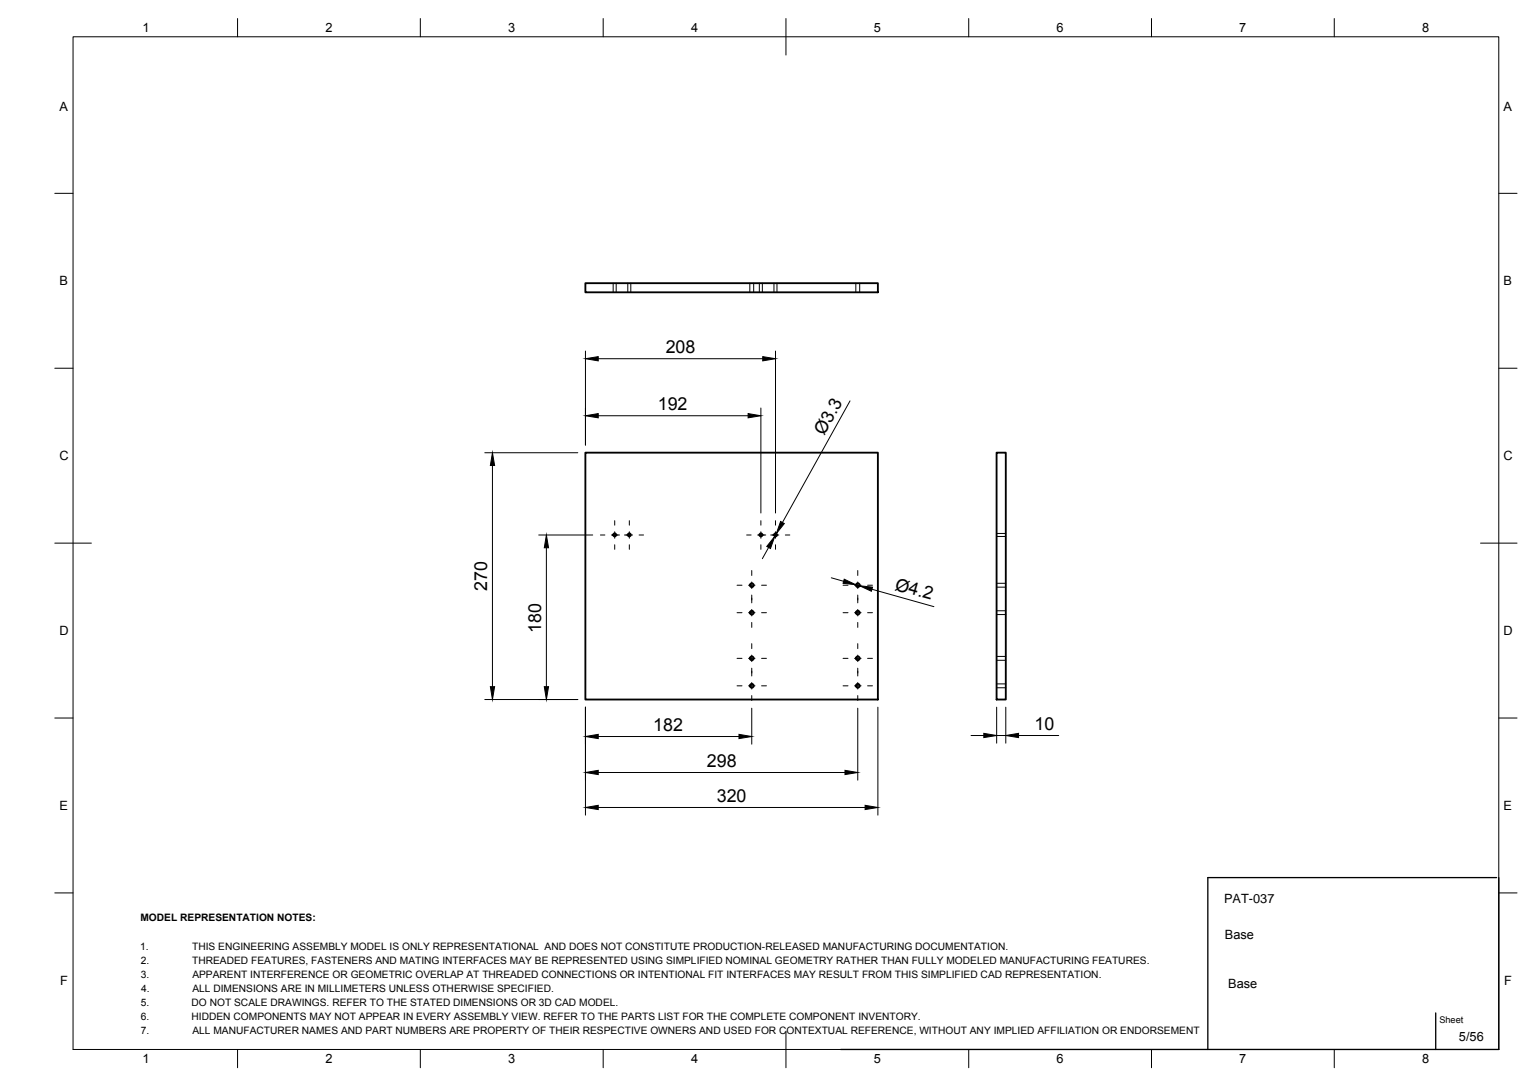
ISO-10303-21;
HEADER;
/* Generated by software containing ST-Developer
 * from STEP Tools, Inc. (www.steptools.com) 
 */

FILE_DESCRIPTION(
/* description */ ('Flywheel Crank-Slider'),
/* implementation_level */ '2;1');

FILE_NAME(
/* name */ 'Base.step',
/* time_stamp */ '2026-10-28T03:23:13-07:00',
/* author */ (''),
/* organization */ (''),
/* preprocessor_version */ 'ST-DEVELOPER v20.2',
/* originating_system */ 'Autodesk Translation Framework v15.17.0.0',
/* authorisation */ '');

FILE_SCHEMA (('AUTOMOTIVE_DESIGN { 1 0 10303 214 3 1 1 }'));
ENDSEC;

DATA;
#10=MECHANICAL_DESIGN_GEOMETRIC_PRESENTATION_REPRESENTATION('',(#668),#17322);
#564=SHAPE_REPRESENTATION_RELATIONSHIP('SRR','None',#17560,#616);
#616=ADVANCED_BREP_SHAPE_REPRESENTATION('',(#729),#17264);
#668=STYLED_ITEM('',(#17910),#729);
#729=MANIFOLD_SOLID_BREP('Body1',#9046);
#785=FACE_BOUND('',#1872,.T.);
#786=FACE_BOUND('',#1873,.T.);
#787=FACE_BOUND('',#1874,.T.);
#788=FACE_BOUND('',#1875,.T.);
#789=FACE_BOUND('',#1876,.T.);
#790=FACE_BOUND('',#1877,.T.);
#791=FACE_BOUND('',#1878,.T.);
#792=FACE_BOUND('',#1879,.T.);
#793=FACE_BOUND('',#1880,.T.);
#794=FACE_BOUND('',#1881,.T.);
#795=FACE_BOUND('',#1882,.T.);
#796=FACE_BOUND('',#1883,.T.);
#797=FACE_BOUND('',#1885,.T.);
#798=FACE_BOUND('',#1886,.T.);
#799=FACE_BOUND('',#1887,.T.);
#800=FACE_BOUND('',#1888,.T.);
#801=FACE_BOUND('',#1889,.T.);
#802=FACE_BOUND('',#1890,.T.);
#803=FACE_BOUND('',#1891,.T.);
#804=FACE_BOUND('',#1892,.T.);
#805=FACE_BOUND('',#1893,.T.);
#806=FACE_BOUND('',#1894,.T.);
#807=FACE_BOUND('',#1895,.T.);
#808=FACE_BOUND('',#1896,.T.);
#1011=PLANE('',#9724);
#1012=PLANE('',#9725);
#1013=PLANE('',#9726);
#1014=PLANE('',#9727);
#1015=PLANE('',#9728);
#1016=PLANE('',#9729);
#1320=FACE_OUTER_BOUND('',#1855,.T.);
#1321=FACE_OUTER_BOUND('',#1856,.T.);
#1322=FACE_OUTER_BOUND('',#1857,.T.);
#1323=FACE_OUTER_BOUND('',#1858,.T.);
#1324=FACE_OUTER_BOUND('',#1859,.T.);
#1325=FACE_OUTER_BOUND('',#1860,.T.);
#1326=FACE_OUTER_BOUND('',#1861,.T.);
#1327=FACE_OUTER_BOUND('',#1862,.T.);
#1328=FACE_OUTER_BOUND('',#1863,.T.);
#1329=FACE_OUTER_BOUND('',#1864,.T.);
#1330=FACE_OUTER_BOUND('',#1865,.T.);
#1331=FACE_OUTER_BOUND('',#1866,.T.);
#1332=FACE_OUTER_BOUND('',#1867,.T.);
#1333=FACE_OUTER_BOUND('',#1868,.T.);
#1334=FACE_OUTER_BOUND('',#1869,.T.);
#1335=FACE_OUTER_BOUND('',#1870,.T.);
#1336=FACE_OUTER_BOUND('',#1871,.T.);
#1337=FACE_OUTER_BOUND('',#1884,.T.);
#1855=EDGE_LOOP('',(#6122,#6123,#6124,#6125));
#1856=EDGE_LOOP('',(#6126,#6127,#6128,#6129));
#1857=EDGE_LOOP('',(#6130,#6131,#6132,#6133));
#1858=EDGE_LOOP('',(#6134,#6135,#6136,#6137));
#1859=EDGE_LOOP('',(#6138,#6139,#6140,#6141));
#1860=EDGE_LOOP('',(#6142,#6143,#6144,#6145));
#1861=EDGE_LOOP('',(#6146,#6147,#6148,#6149));
#1862=EDGE_LOOP('',(#6150,#6151,#6152,#6153));
#1863=EDGE_LOOP('',(#6154,#6155,#6156,#6157));
#1864=EDGE_LOOP('',(#6158,#6159,#6160,#6161));
#1865=EDGE_LOOP('',(#6162,#6163,#6164,#6165));
#1866=EDGE_LOOP('',(#6166,#6167,#6168,#6169));
#1867=EDGE_LOOP('',(#6170,#6171,#6172,#6173));
#1868=EDGE_LOOP('',(#6174,#6175,#6176,#6177));
#1869=EDGE_LOOP('',(#6178,#6179,#6180,#6181));
#1870=EDGE_LOOP('',(#6182,#6183,#6184,#6185));
#1871=EDGE_LOOP('',(#6186,#6187,#6188,#6189));
#1872=EDGE_LOOP('',(#6190));
#1873=EDGE_LOOP('',(#6191));
#1874=EDGE_LOOP('',(#6192));
#1875=EDGE_LOOP('',(#6193));
#1876=EDGE_LOOP('',(#6194));
#1877=EDGE_LOOP('',(#6195));
#1878=EDGE_LOOP('',(#6196));
#1879=EDGE_LOOP('',(#6197));
#1880=EDGE_LOOP('',(#6198));
#1881=EDGE_LOOP('',(#6199));
#1882=EDGE_LOOP('',(#6200));
#1883=EDGE_LOOP('',(#6201));
#1884=EDGE_LOOP('',(#6202,#6203,#6204,#6205));
#1885=EDGE_LOOP('',(#6206));
#1886=EDGE_LOOP('',(#6207));
#1887=EDGE_LOOP('',(#6208));
#1888=EDGE_LOOP('',(#6209));
#1889=EDGE_LOOP('',(#6210));
#1890=EDGE_LOOP('',(#6211));
#1891=EDGE_LOOP('',(#6212));
#1892=EDGE_LOOP('',(#6213));
#1893=EDGE_LOOP('',(#6214));
#1894=EDGE_LOOP('',(#6215));
#1895=EDGE_LOOP('',(#6216));
#1896=EDGE_LOOP('',(#6217));
#2616=LINE('',#13738,#3227);
#2617=LINE('',#13744,#3228);
#2618=LINE('',#13750,#3229);
#2619=LINE('',#13756,#3230);
#2620=LINE('',#13762,#3231);
#2621=LINE('',#13768,#3232);
#2622=LINE('',#13774,#3233);
#2623=LINE('',#13780,#3234);
#2624=LINE('',#13786,#3235);
#2625=LINE('',#13792,#3236);
#2626=LINE('',#13798,#3237);
#2627=LINE('',#13804,#3238);
#2628=LINE('',#13809,#3239);
#2629=LINE('',#13811,#3240);
#2630=LINE('',#13813,#3241);
#2631=LINE('',#13814,#3242);
#2632=LINE('',#13817,#3243);
#2633=LINE('',#13819,#3244);
#2634=LINE('',#13820,#3245);
#2635=LINE('',#13823,#3246);
#2636=LINE('',#13825,#3247);
#2637=LINE('',#13826,#3248);
#2638=LINE('',#13828,#3249);
#2639=LINE('',#13829,#3250);
#3227=VECTOR('',#10840,0.164999999999999);
#3228=VECTOR('',#10847,0.164999999999999);
#3229=VECTOR('',#10854,0.165);
#3230=VECTOR('',#10861,0.165);
#3231=VECTOR('',#10868,0.21);
#3232=VECTOR('',#10875,0.21);
#3233=VECTOR('',#10882,0.21);
#3234=VECTOR('',#10889,0.21);
#3235=VECTOR('',#10896,0.21);
#3236=VECTOR('',#10903,0.21);
#3237=VECTOR('',#10910,0.21);
#3238=VECTOR('',#10917,0.21);
#3239=VECTOR('',#10922,1.);
#3240=VECTOR('',#10923,1.);
#3241=VECTOR('',#10924,1.);
#3242=VECTOR('',#10925,1.);
#3243=VECTOR('',#10928,1.);
#3244=VECTOR('',#10929,1.);
#3245=VECTOR('',#10930,1.);
#3246=VECTOR('',#10933,1.);
#3247=VECTOR('',#10934,1.);
#3248=VECTOR('',#10935,1.);
#3249=VECTOR('',#10938,1.);
#3250=VECTOR('',#10939,1.);
#3838=CIRCLE('',#9689,0.164999999999999);
#3839=CIRCLE('',#9690,0.164999999999999);
#3840=CIRCLE('',#9692,0.164999999999999);
#3841=CIRCLE('',#9693,0.164999999999999);
#3842=CIRCLE('',#9695,0.165);
#3843=CIRCLE('',#9696,0.165);
#3844=CIRCLE('',#9698,0.165);
#3845=CIRCLE('',#9699,0.165);
#3846=CIRCLE('',#9701,0.21);
#3847=CIRCLE('',#9702,0.21);
#3848=CIRCLE('',#9704,0.21);
#3849=CIRCLE('',#9705,0.21);
#3850=CIRCLE('',#9707,0.21);
#3851=CIRCLE('',#9708,0.21);
#3852=CIRCLE('',#9710,0.21);
#3853=CIRCLE('',#9711,0.21);
#3854=CIRCLE('',#9713,0.21);
#3855=CIRCLE('',#9714,0.21);
#3856=CIRCLE('',#9716,0.21);
#3857=CIRCLE('',#9717,0.21);
#3858=CIRCLE('',#9719,0.21);
#3859=CIRCLE('',#9720,0.21);
#3860=CIRCLE('',#9722,0.21);
#3861=CIRCLE('',#9723,0.21);
#4277=VERTEX_POINT('',#13735);
#4278=VERTEX_POINT('',#13737);
#4279=VERTEX_POINT('',#13741);
#4280=VERTEX_POINT('',#13743);
#4281=VERTEX_POINT('',#13747);
#4282=VERTEX_POINT('',#13749);
#4283=VERTEX_POINT('',#13753);
#4284=VERTEX_POINT('',#13755);
#4285=VERTEX_POINT('',#13759);
#4286=VERTEX_POINT('',#13761);
#4287=VERTEX_POINT('',#13765);
#4288=VERTEX_POINT('',#13767);
#4289=VERTEX_POINT('',#13771);
#4290=VERTEX_POINT('',#13773);
#4291=VERTEX_POINT('',#13777);
#4292=VERTEX_POINT('',#13779);
#4293=VERTEX_POINT('',#13783);
#4294=VERTEX_POINT('',#13785);
#4295=VERTEX_POINT('',#13789);
#4296=VERTEX_POINT('',#13791);
#4297=VERTEX_POINT('',#13795);
#4298=VERTEX_POINT('',#13797);
#4299=VERTEX_POINT('',#13801);
#4300=VERTEX_POINT('',#13803);
#4301=VERTEX_POINT('',#13807);
#4302=VERTEX_POINT('',#13808);
#4303=VERTEX_POINT('',#13810);
#4304=VERTEX_POINT('',#13812);
#4305=VERTEX_POINT('',#13816);
#4306=VERTEX_POINT('',#13818);
#4307=VERTEX_POINT('',#13822);
#4308=VERTEX_POINT('',#13824);
#5018=EDGE_CURVE('',#4277,#4277,#3838,.T.);
#5019=EDGE_CURVE('',#4277,#4278,#2616,.T.);
#5020=EDGE_CURVE('',#4278,#4278,#3839,.T.);
#5021=EDGE_CURVE('',#4279,#4279,#3840,.T.);
#5022=EDGE_CURVE('',#4279,#4280,#2617,.T.);
#5023=EDGE_CURVE('',#4280,#4280,#3841,.T.);
#5024=EDGE_CURVE('',#4281,#4281,#3842,.T.);
#5025=EDGE_CURVE('',#4281,#4282,#2618,.T.);
#5026=EDGE_CURVE('',#4282,#4282,#3843,.T.);
#5027=EDGE_CURVE('',#4283,#4283,#3844,.T.);
#5028=EDGE_CURVE('',#4283,#4284,#2619,.T.);
#5029=EDGE_CURVE('',#4284,#4284,#3845,.T.);
#5030=EDGE_CURVE('',#4285,#4285,#3846,.T.);
#5031=EDGE_CURVE('',#4285,#4286,#2620,.T.);
#5032=EDGE_CURVE('',#4286,#4286,#3847,.T.);
#5033=EDGE_CURVE('',#4287,#4287,#3848,.T.);
#5034=EDGE_CURVE('',#4287,#4288,#2621,.T.);
#5035=EDGE_CURVE('',#4288,#4288,#3849,.T.);
#5036=EDGE_CURVE('',#4289,#4289,#3850,.T.);
#5037=EDGE_CURVE('',#4289,#4290,#2622,.T.);
#5038=EDGE_CURVE('',#4290,#4290,#3851,.T.);
#5039=EDGE_CURVE('',#4291,#4291,#3852,.T.);
#5040=EDGE_CURVE('',#4291,#4292,#2623,.T.);
#5041=EDGE_CURVE('',#4292,#4292,#3853,.T.);
#5042=EDGE_CURVE('',#4293,#4293,#3854,.T.);
#5043=EDGE_CURVE('',#4293,#4294,#2624,.T.);
#5044=EDGE_CURVE('',#4294,#4294,#3855,.T.);
#5045=EDGE_CURVE('',#4295,#4295,#3856,.T.);
#5046=EDGE_CURVE('',#4295,#4296,#2625,.T.);
#5047=EDGE_CURVE('',#4296,#4296,#3857,.T.);
#5048=EDGE_CURVE('',#4297,#4297,#3858,.T.);
#5049=EDGE_CURVE('',#4297,#4298,#2626,.T.);
#5050=EDGE_CURVE('',#4298,#4298,#3859,.T.);
#5051=EDGE_CURVE('',#4299,#4299,#3860,.T.);
#5052=EDGE_CURVE('',#4299,#4300,#2627,.T.);
#5053=EDGE_CURVE('',#4300,#4300,#3861,.T.);
#5054=EDGE_CURVE('',#4301,#4302,#2628,.T.);
#5055=EDGE_CURVE('',#4302,#4303,#2629,.T.);
#5056=EDGE_CURVE('',#4304,#4303,#2630,.T.);
#5057=EDGE_CURVE('',#4301,#4304,#2631,.T.);
#5058=EDGE_CURVE('',#4305,#4301,#2632,.T.);
#5059=EDGE_CURVE('',#4306,#4304,#2633,.T.);
#5060=EDGE_CURVE('',#4305,#4306,#2634,.T.);
#5061=EDGE_CURVE('',#4307,#4305,#2635,.T.);
#5062=EDGE_CURVE('',#4308,#4306,#2636,.T.);
#5063=EDGE_CURVE('',#4307,#4308,#2637,.T.);
#5064=EDGE_CURVE('',#4302,#4307,#2638,.T.);
#5065=EDGE_CURVE('',#4303,#4308,#2639,.T.);
#6122=ORIENTED_EDGE('',*,*,#5018,.F.);
#6123=ORIENTED_EDGE('',*,*,#5019,.T.);
#6124=ORIENTED_EDGE('',*,*,#5020,.F.);
#6125=ORIENTED_EDGE('',*,*,#5019,.F.);
#6126=ORIENTED_EDGE('',*,*,#5021,.F.);
#6127=ORIENTED_EDGE('',*,*,#5022,.T.);
#6128=ORIENTED_EDGE('',*,*,#5023,.F.);
#6129=ORIENTED_EDGE('',*,*,#5022,.F.);
#6130=ORIENTED_EDGE('',*,*,#5024,.F.);
#6131=ORIENTED_EDGE('',*,*,#5025,.T.);
#6132=ORIENTED_EDGE('',*,*,#5026,.F.);
#6133=ORIENTED_EDGE('',*,*,#5025,.F.);
#6134=ORIENTED_EDGE('',*,*,#5027,.F.);
#6135=ORIENTED_EDGE('',*,*,#5028,.T.);
#6136=ORIENTED_EDGE('',*,*,#5029,.F.);
#6137=ORIENTED_EDGE('',*,*,#5028,.F.);
#6138=ORIENTED_EDGE('',*,*,#5030,.F.);
#6139=ORIENTED_EDGE('',*,*,#5031,.T.);
#6140=ORIENTED_EDGE('',*,*,#5032,.F.);
#6141=ORIENTED_EDGE('',*,*,#5031,.F.);
#6142=ORIENTED_EDGE('',*,*,#5033,.F.);
#6143=ORIENTED_EDGE('',*,*,#5034,.T.);
#6144=ORIENTED_EDGE('',*,*,#5035,.F.);
#6145=ORIENTED_EDGE('',*,*,#5034,.F.);
#6146=ORIENTED_EDGE('',*,*,#5036,.F.);
#6147=ORIENTED_EDGE('',*,*,#5037,.T.);
#6148=ORIENTED_EDGE('',*,*,#5038,.F.);
#6149=ORIENTED_EDGE('',*,*,#5037,.F.);
#6150=ORIENTED_EDGE('',*,*,#5039,.F.);
#6151=ORIENTED_EDGE('',*,*,#5040,.T.);
#6152=ORIENTED_EDGE('',*,*,#5041,.F.);
#6153=ORIENTED_EDGE('',*,*,#5040,.F.);
#6154=ORIENTED_EDGE('',*,*,#5042,.F.);
#6155=ORIENTED_EDGE('',*,*,#5043,.T.);
#6156=ORIENTED_EDGE('',*,*,#5044,.F.);
#6157=ORIENTED_EDGE('',*,*,#5043,.F.);
#6158=ORIENTED_EDGE('',*,*,#5045,.F.);
#6159=ORIENTED_EDGE('',*,*,#5046,.T.);
#6160=ORIENTED_EDGE('',*,*,#5047,.F.);
#6161=ORIENTED_EDGE('',*,*,#5046,.F.);
#6162=ORIENTED_EDGE('',*,*,#5048,.F.);
#6163=ORIENTED_EDGE('',*,*,#5049,.T.);
#6164=ORIENTED_EDGE('',*,*,#5050,.F.);
#6165=ORIENTED_EDGE('',*,*,#5049,.F.);
#6166=ORIENTED_EDGE('',*,*,#5051,.F.);
#6167=ORIENTED_EDGE('',*,*,#5052,.T.);
#6168=ORIENTED_EDGE('',*,*,#5053,.F.);
#6169=ORIENTED_EDGE('',*,*,#5052,.F.);
#6170=ORIENTED_EDGE('',*,*,#5054,.T.);
#6171=ORIENTED_EDGE('',*,*,#5055,.T.);
#6172=ORIENTED_EDGE('',*,*,#5056,.F.);
#6173=ORIENTED_EDGE('',*,*,#5057,.F.);
#6174=ORIENTED_EDGE('',*,*,#5058,.T.);
#6175=ORIENTED_EDGE('',*,*,#5057,.T.);
#6176=ORIENTED_EDGE('',*,*,#5059,.F.);
#6177=ORIENTED_EDGE('',*,*,#5060,.F.);
#6178=ORIENTED_EDGE('',*,*,#5061,.T.);
#6179=ORIENTED_EDGE('',*,*,#5060,.T.);
#6180=ORIENTED_EDGE('',*,*,#5062,.F.);
#6181=ORIENTED_EDGE('',*,*,#5063,.F.);
#6182=ORIENTED_EDGE('',*,*,#5064,.T.);
#6183=ORIENTED_EDGE('',*,*,#5063,.T.);
#6184=ORIENTED_EDGE('',*,*,#5065,.F.);
#6185=ORIENTED_EDGE('',*,*,#5055,.F.);
#6186=ORIENTED_EDGE('',*,*,#5065,.T.);
#6187=ORIENTED_EDGE('',*,*,#5062,.T.);
#6188=ORIENTED_EDGE('',*,*,#5059,.T.);
#6189=ORIENTED_EDGE('',*,*,#5056,.T.);
#6190=ORIENTED_EDGE('',*,*,#5026,.T.);
#6191=ORIENTED_EDGE('',*,*,#5029,.T.);
#6192=ORIENTED_EDGE('',*,*,#5053,.T.);
#6193=ORIENTED_EDGE('',*,*,#5050,.T.);
#6194=ORIENTED_EDGE('',*,*,#5047,.T.);
#6195=ORIENTED_EDGE('',*,*,#5044,.T.);
#6196=ORIENTED_EDGE('',*,*,#5041,.T.);
#6197=ORIENTED_EDGE('',*,*,#5038,.T.);
#6198=ORIENTED_EDGE('',*,*,#5035,.T.);
#6199=ORIENTED_EDGE('',*,*,#5032,.T.);
#6200=ORIENTED_EDGE('',*,*,#5023,.T.);
#6201=ORIENTED_EDGE('',*,*,#5020,.T.);
#6202=ORIENTED_EDGE('',*,*,#5064,.F.);
#6203=ORIENTED_EDGE('',*,*,#5054,.F.);
#6204=ORIENTED_EDGE('',*,*,#5058,.F.);
#6205=ORIENTED_EDGE('',*,*,#5061,.F.);
#6206=ORIENTED_EDGE('',*,*,#5024,.T.);
#6207=ORIENTED_EDGE('',*,*,#5027,.T.);
#6208=ORIENTED_EDGE('',*,*,#5051,.T.);
#6209=ORIENTED_EDGE('',*,*,#5048,.T.);
#6210=ORIENTED_EDGE('',*,*,#5045,.T.);
#6211=ORIENTED_EDGE('',*,*,#5042,.T.);
#6212=ORIENTED_EDGE('',*,*,#5039,.T.);
#6213=ORIENTED_EDGE('',*,*,#5036,.T.);
#6214=ORIENTED_EDGE('',*,*,#5033,.T.);
#6215=ORIENTED_EDGE('',*,*,#5030,.T.);
#6216=ORIENTED_EDGE('',*,*,#5021,.T.);
#6217=ORIENTED_EDGE('',*,*,#5018,.T.);
#8330=CYLINDRICAL_SURFACE('',#9688,0.164999999999999);
#8331=CYLINDRICAL_SURFACE('',#9691,0.164999999999999);
#8332=CYLINDRICAL_SURFACE('',#9694,0.165);
#8333=CYLINDRICAL_SURFACE('',#9697,0.165);
#8334=CYLINDRICAL_SURFACE('',#9700,0.21);
#8335=CYLINDRICAL_SURFACE('',#9703,0.21);
#8336=CYLINDRICAL_SURFACE('',#9706,0.21);
#8337=CYLINDRICAL_SURFACE('',#9709,0.21);
#8338=CYLINDRICAL_SURFACE('',#9712,0.21);
#8339=CYLINDRICAL_SURFACE('',#9715,0.21);
#8340=CYLINDRICAL_SURFACE('',#9718,0.21);
#8341=CYLINDRICAL_SURFACE('',#9721,0.21);
#8511=ADVANCED_FACE('',(#1320),#8330,.F.);
#8512=ADVANCED_FACE('',(#1321),#8331,.F.);
#8513=ADVANCED_FACE('',(#1322),#8332,.F.);
#8514=ADVANCED_FACE('',(#1323),#8333,.F.);
#8515=ADVANCED_FACE('',(#1324),#8334,.F.);
#8516=ADVANCED_FACE('',(#1325),#8335,.F.);
#8517=ADVANCED_FACE('',(#1326),#8336,.F.);
#8518=ADVANCED_FACE('',(#1327),#8337,.F.);
#8519=ADVANCED_FACE('',(#1328),#8338,.F.);
#8520=ADVANCED_FACE('',(#1329),#8339,.F.);
#8521=ADVANCED_FACE('',(#1330),#8340,.F.);
#8522=ADVANCED_FACE('',(#1331),#8341,.F.);
#8523=ADVANCED_FACE('',(#1332),#1011,.T.);
#8524=ADVANCED_FACE('',(#1333),#1012,.T.);
#8525=ADVANCED_FACE('',(#1334),#1013,.T.);
#8526=ADVANCED_FACE('',(#1335),#1014,.T.);
#8527=ADVANCED_FACE('',(#1336,#785,#786,#787,#788,#789,#790,#791,#792,#793,
#794,#795,#796),#1015,.T.);
#8528=ADVANCED_FACE('',(#1337,#797,#798,#799,#800,#801,#802,#803,#804,#805,
#806,#807,#808),#1016,.F.);
#9046=CLOSED_SHELL('',(#8511,#8512,#8513,#8514,#8515,#8516,#8517,#8518,
#8519,#8520,#8521,#8522,#8523,#8524,#8525,#8526,#8527,#8528));
#9687=AXIS2_PLACEMENT_3D('',#13733,#10834,#10835);
#9688=AXIS2_PLACEMENT_3D('',#13734,#10836,#10837);
#9689=AXIS2_PLACEMENT_3D('',#13736,#10838,#10839);
#9690=AXIS2_PLACEMENT_3D('',#13739,#10841,#10842);
#9691=AXIS2_PLACEMENT_3D('',#13740,#10843,#10844);
#9692=AXIS2_PLACEMENT_3D('',#13742,#10845,#10846);
#9693=AXIS2_PLACEMENT_3D('',#13745,#10848,#10849);
#9694=AXIS2_PLACEMENT_3D('',#13746,#10850,#10851);
#9695=AXIS2_PLACEMENT_3D('',#13748,#10852,#10853);
#9696=AXIS2_PLACEMENT_3D('',#13751,#10855,#10856);
#9697=AXIS2_PLACEMENT_3D('',#13752,#10857,#10858);
#9698=AXIS2_PLACEMENT_3D('',#13754,#10859,#10860);
#9699=AXIS2_PLACEMENT_3D('',#13757,#10862,#10863);
#9700=AXIS2_PLACEMENT_3D('',#13758,#10864,#10865);
#9701=AXIS2_PLACEMENT_3D('',#13760,#10866,#10867);
#9702=AXIS2_PLACEMENT_3D('',#13763,#10869,#10870);
#9703=AXIS2_PLACEMENT_3D('',#13764,#10871,#10872);
#9704=AXIS2_PLACEMENT_3D('',#13766,#10873,#10874);
#9705=AXIS2_PLACEMENT_3D('',#13769,#10876,#10877);
#9706=AXIS2_PLACEMENT_3D('',#13770,#10878,#10879);
#9707=AXIS2_PLACEMENT_3D('',#13772,#10880,#10881);
#9708=AXIS2_PLACEMENT_3D('',#13775,#10883,#10884);
#9709=AXIS2_PLACEMENT_3D('',#13776,#10885,#10886);
#9710=AXIS2_PLACEMENT_3D('',#13778,#10887,#10888);
#9711=AXIS2_PLACEMENT_3D('',#13781,#10890,#10891);
#9712=AXIS2_PLACEMENT_3D('',#13782,#10892,#10893);
#9713=AXIS2_PLACEMENT_3D('',#13784,#10894,#10895);
#9714=AXIS2_PLACEMENT_3D('',#13787,#10897,#10898);
#9715=AXIS2_PLACEMENT_3D('',#13788,#10899,#10900);
#9716=AXIS2_PLACEMENT_3D('',#13790,#10901,#10902);
#9717=AXIS2_PLACEMENT_3D('',#13793,#10904,#10905);
#9718=AXIS2_PLACEMENT_3D('',#13794,#10906,#10907);
#9719=AXIS2_PLACEMENT_3D('',#13796,#10908,#10909);
#9720=AXIS2_PLACEMENT_3D('',#13799,#10911,#10912);
#9721=AXIS2_PLACEMENT_3D('',#13800,#10913,#10914);
#9722=AXIS2_PLACEMENT_3D('',#13802,#10915,#10916);
#9723=AXIS2_PLACEMENT_3D('',#13805,#10918,#10919);
#9724=AXIS2_PLACEMENT_3D('',#13806,#10920,#10921);
#9725=AXIS2_PLACEMENT_3D('',#13815,#10926,#10927);
#9726=AXIS2_PLACEMENT_3D('',#13821,#10931,#10932);
#9727=AXIS2_PLACEMENT_3D('',#13827,#10936,#10937);
#9728=AXIS2_PLACEMENT_3D('',#13830,#10940,#10941);
#9729=AXIS2_PLACEMENT_3D('',#13831,#10942,#10943);
#10834=DIRECTION('axis',(0.,0.,1.));
#10835=DIRECTION('refdir',(1.,0.,0.));
#10836=DIRECTION('center_axis',(0.,0.,1.));
#10837=DIRECTION('ref_axis',(1.,0.,0.));
#10838=DIRECTION('center_axis',(0.,0.,1.));
#10839=DIRECTION('ref_axis',(1.,0.,0.));
#10840=DIRECTION('',(0.,0.,1.));
#10841=DIRECTION('center_axis',(0.,0.,-1.));
#10842=DIRECTION('ref_axis',(1.,0.,0.));
#10843=DIRECTION('center_axis',(0.,0.,1.));
#10844=DIRECTION('ref_axis',(1.,0.,0.));
#10845=DIRECTION('center_axis',(0.,0.,1.));
#10846=DIRECTION('ref_axis',(1.,0.,0.));
#10847=DIRECTION('',(0.,0.,1.));
#10848=DIRECTION('center_axis',(0.,0.,-1.));
#10849=DIRECTION('ref_axis',(1.,0.,0.));
#10850=DIRECTION('center_axis',(0.,0.,1.));
#10851=DIRECTION('ref_axis',(1.,0.,0.));
#10852=DIRECTION('center_axis',(0.,0.,1.));
#10853=DIRECTION('ref_axis',(1.,0.,0.));
#10854=DIRECTION('',(0.,0.,1.));
#10855=DIRECTION('center_axis',(0.,0.,-1.));
#10856=DIRECTION('ref_axis',(1.,0.,0.));
#10857=DIRECTION('center_axis',(0.,0.,1.));
#10858=DIRECTION('ref_axis',(1.,0.,0.));
#10859=DIRECTION('center_axis',(0.,0.,1.));
#10860=DIRECTION('ref_axis',(1.,0.,0.));
#10861=DIRECTION('',(0.,0.,1.));
#10862=DIRECTION('center_axis',(0.,0.,-1.));
#10863=DIRECTION('ref_axis',(1.,0.,0.));
#10864=DIRECTION('center_axis',(0.,0.,1.));
#10865=DIRECTION('ref_axis',(1.,0.,0.));
#10866=DIRECTION('center_axis',(0.,0.,1.));
#10867=DIRECTION('ref_axis',(1.,0.,0.));
#10868=DIRECTION('',(0.,0.,1.));
#10869=DIRECTION('center_axis',(0.,0.,-1.));
#10870=DIRECTION('ref_axis',(1.,0.,0.));
#10871=DIRECTION('center_axis',(0.,0.,1.));
#10872=DIRECTION('ref_axis',(1.,0.,0.));
#10873=DIRECTION('center_axis',(0.,0.,1.));
#10874=DIRECTION('ref_axis',(1.,0.,0.));
#10875=DIRECTION('',(0.,0.,1.));
#10876=DIRECTION('center_axis',(0.,0.,-1.));
#10877=DIRECTION('ref_axis',(1.,0.,0.));
#10878=DIRECTION('center_axis',(0.,0.,1.));
#10879=DIRECTION('ref_axis',(1.,0.,0.));
#10880=DIRECTION('center_axis',(0.,0.,1.));
#10881=DIRECTION('ref_axis',(1.,0.,0.));
#10882=DIRECTION('',(0.,0.,1.));
#10883=DIRECTION('center_axis',(0.,0.,-1.));
#10884=DIRECTION('ref_axis',(1.,0.,0.));
#10885=DIRECTION('center_axis',(0.,0.,1.));
#10886=DIRECTION('ref_axis',(1.,0.,0.));
#10887=DIRECTION('center_axis',(0.,0.,1.));
#10888=DIRECTION('ref_axis',(1.,0.,0.));
#10889=DIRECTION('',(0.,0.,1.));
#10890=DIRECTION('center_axis',(0.,0.,-1.));
#10891=DIRECTION('ref_axis',(1.,0.,0.));
#10892=DIRECTION('center_axis',(0.,0.,1.));
#10893=DIRECTION('ref_axis',(1.,0.,0.));
#10894=DIRECTION('center_axis',(0.,0.,1.));
#10895=DIRECTION('ref_axis',(1.,0.,0.));
#10896=DIRECTION('',(0.,0.,1.));
#10897=DIRECTION('center_axis',(0.,0.,-1.));
#10898=DIRECTION('ref_axis',(1.,0.,0.));
#10899=DIRECTION('center_axis',(0.,0.,1.));
#10900=DIRECTION('ref_axis',(1.,0.,0.));
#10901=DIRECTION('center_axis',(0.,0.,1.));
#10902=DIRECTION('ref_axis',(1.,0.,0.));
#10903=DIRECTION('',(0.,0.,1.));
#10904=DIRECTION('center_axis',(0.,0.,-1.));
#10905=DIRECTION('ref_axis',(1.,0.,0.));
#10906=DIRECTION('center_axis',(0.,0.,1.));
#10907=DIRECTION('ref_axis',(1.,0.,0.));
#10908=DIRECTION('center_axis',(0.,0.,1.));
#10909=DIRECTION('ref_axis',(1.,0.,0.));
#10910=DIRECTION('',(0.,0.,1.));
#10911=DIRECTION('center_axis',(0.,0.,-1.));
#10912=DIRECTION('ref_axis',(1.,0.,0.));
#10913=DIRECTION('center_axis',(0.,0.,1.));
#10914=DIRECTION('ref_axis',(1.,0.,0.));
#10915=DIRECTION('center_axis',(0.,0.,1.));
#10916=DIRECTION('ref_axis',(1.,0.,0.));
#10917=DIRECTION('',(0.,0.,1.));
#10918=DIRECTION('center_axis',(0.,0.,-1.));
#10919=DIRECTION('ref_axis',(1.,0.,0.));
#10920=DIRECTION('center_axis',(0.,1.,0.));
#10921=DIRECTION('ref_axis',(-1.,0.,0.));
#10922=DIRECTION('',(-1.,0.,0.));
#10923=DIRECTION('',(0.,0.,1.));
#10924=DIRECTION('',(-1.,0.,0.));
#10925=DIRECTION('',(0.,0.,1.));
#10926=DIRECTION('center_axis',(1.,0.,0.));
#10927=DIRECTION('ref_axis',(0.,1.,0.));
#10928=DIRECTION('',(0.,1.,0.));
#10929=DIRECTION('',(0.,1.,0.));
#10930=DIRECTION('',(0.,0.,1.));
#10931=DIRECTION('center_axis',(0.,-1.,0.));
#10932=DIRECTION('ref_axis',(1.,0.,0.));
#10933=DIRECTION('',(1.,0.,0.));
#10934=DIRECTION('',(1.,0.,0.));
#10935=DIRECTION('',(0.,0.,1.));
#10936=DIRECTION('center_axis',(-1.,0.,0.));
#10937=DIRECTION('ref_axis',(0.,-1.,0.));
#10938=DIRECTION('',(0.,-1.,0.));
#10939=DIRECTION('',(0.,-1.,0.));
#10940=DIRECTION('center_axis',(0.,0.,1.));
#10941=DIRECTION('ref_axis',(1.,0.,0.));
#10942=DIRECTION('center_axis',(0.,0.,1.));
#10943=DIRECTION('ref_axis',(1.,0.,0.));
#13733=CARTESIAN_POINT('',(0.,0.,0.));
#13734=CARTESIAN_POINT('Origin',(19.2,0.,-0.1));
#13735=CARTESIAN_POINT('',(19.035,-2.02066721859312E-17,0.));
#13736=CARTESIAN_POINT('Origin',(19.2,0.,0.));
#13737=CARTESIAN_POINT('',(19.035,2.02066721859312E-17,1.));
#13738=CARTESIAN_POINT('',(19.035,-2.02066721859312E-17,-0.1));
#13739=CARTESIAN_POINT('Origin',(19.2,0.,1.));
#13740=CARTESIAN_POINT('Origin',(20.8,0.,-0.1));
#13741=CARTESIAN_POINT('',(20.635,-2.02066721859312E-17,0.));
#13742=CARTESIAN_POINT('Origin',(20.8,0.,0.));
#13743=CARTESIAN_POINT('',(20.635,2.02066721859312E-17,1.));
#13744=CARTESIAN_POINT('',(20.635,-2.02066721859312E-17,-0.1));
#13745=CARTESIAN_POINT('Origin',(20.8,0.,1.));
#13746=CARTESIAN_POINT('Origin',(3.2,0.,-0.1));
#13747=CARTESIAN_POINT('',(3.035,-2.02066721859313E-17,0.));
#13748=CARTESIAN_POINT('Origin',(3.2,0.,0.));
#13749=CARTESIAN_POINT('',(3.035,2.02066721859313E-17,1.));
#13750=CARTESIAN_POINT('',(3.035,-2.02066721859313E-17,-0.1));
#13751=CARTESIAN_POINT('Origin',(3.2,0.,1.));
#13752=CARTESIAN_POINT('Origin',(4.8,0.,-0.1));
#13753=CARTESIAN_POINT('',(4.635,-2.02066721859313E-17,0.));
#13754=CARTESIAN_POINT('Origin',(4.8,0.,0.));
#13755=CARTESIAN_POINT('',(4.635,2.02066721859313E-17,1.));
#13756=CARTESIAN_POINT('',(4.635,-2.02066721859313E-17,-0.1));
#13757=CARTESIAN_POINT('Origin',(4.8,0.,1.));
#13758=CARTESIAN_POINT('Origin',(5.8,-8.5,-0.1));
#13759=CARTESIAN_POINT('',(5.59,-8.5,0.));
#13760=CARTESIAN_POINT('Origin',(5.8,-8.5,0.));
#13761=CARTESIAN_POINT('',(5.59,-8.5,1.));
#13762=CARTESIAN_POINT('',(5.59,-8.5,-0.1));
#13763=CARTESIAN_POINT('Origin',(5.8,-8.5,1.));
#13764=CARTESIAN_POINT('Origin',(-5.8,-5.5,-0.1));
#13765=CARTESIAN_POINT('',(-6.01,-5.5,0.));
#13766=CARTESIAN_POINT('Origin',(-5.8,-5.5,0.));
#13767=CARTESIAN_POINT('',(-6.01,-5.5,1.));
#13768=CARTESIAN_POINT('',(-6.01,-5.5,-0.1));
#13769=CARTESIAN_POINT('Origin',(-5.8,-5.5,1.));
#13770=CARTESIAN_POINT('Origin',(-5.8,-8.5,-0.1));
#13771=CARTESIAN_POINT('',(-6.01,-8.5,0.));
#13772=CARTESIAN_POINT('Origin',(-5.8,-8.5,0.));
#13773=CARTESIAN_POINT('',(-6.01,-8.5,1.));
#13774=CARTESIAN_POINT('',(-6.01,-8.5,-0.1));
#13775=CARTESIAN_POINT('Origin',(-5.8,-8.5,1.));
#13776=CARTESIAN_POINT('Origin',(5.8,-5.5,-0.1));
#13777=CARTESIAN_POINT('',(5.59,-5.5,0.));
#13778=CARTESIAN_POINT('Origin',(5.8,-5.5,0.));
#13779=CARTESIAN_POINT('',(5.59,-5.5,1.));
#13780=CARTESIAN_POINT('',(5.59,-5.5,-0.1));
#13781=CARTESIAN_POINT('Origin',(5.8,-5.5,1.));
#13782=CARTESIAN_POINT('Origin',(5.8,-16.5,-0.1));
#13783=CARTESIAN_POINT('',(5.59,-16.5,0.));
#13784=CARTESIAN_POINT('Origin',(5.8,-16.5,0.));
#13785=CARTESIAN_POINT('',(5.59,-16.5,1.));
#13786=CARTESIAN_POINT('',(5.59,-16.5,-0.1));
#13787=CARTESIAN_POINT('Origin',(5.8,-16.5,1.));
#13788=CARTESIAN_POINT('Origin',(-5.8,-13.5,-0.1));
#13789=CARTESIAN_POINT('',(-6.01,-13.5,0.));
#13790=CARTESIAN_POINT('Origin',(-5.8,-13.5,0.));
#13791=CARTESIAN_POINT('',(-6.01,-13.5,1.));
#13792=CARTESIAN_POINT('',(-6.01,-13.5,-0.1));
#13793=CARTESIAN_POINT('Origin',(-5.8,-13.5,1.));
#13794=CARTESIAN_POINT('Origin',(-5.8,-16.5,-0.1));
#13795=CARTESIAN_POINT('',(-6.01,-16.5,0.));
#13796=CARTESIAN_POINT('Origin',(-5.8,-16.5,0.));
#13797=CARTESIAN_POINT('',(-6.01,-16.5,1.));
#13798=CARTESIAN_POINT('',(-6.01,-16.5,-0.1));
#13799=CARTESIAN_POINT('Origin',(-5.8,-16.5,1.));
#13800=CARTESIAN_POINT('Origin',(5.8,-13.5,-0.1));
#13801=CARTESIAN_POINT('',(5.59,-13.5,0.));
#13802=CARTESIAN_POINT('Origin',(5.8,-13.5,0.));
#13803=CARTESIAN_POINT('',(5.59,-13.5,1.));
#13804=CARTESIAN_POINT('',(5.59,-13.5,-0.1));
#13805=CARTESIAN_POINT('Origin',(5.8,-13.5,1.));
#13806=CARTESIAN_POINT('Origin',(24.,9.,0.));
#13807=CARTESIAN_POINT('',(24.,9.,0.));
#13808=CARTESIAN_POINT('',(-8.,9.,0.));
#13809=CARTESIAN_POINT('',(24.,9.,0.));
#13810=CARTESIAN_POINT('',(-8.,9.,1.));
#13811=CARTESIAN_POINT('',(-8.,9.,0.));
#13812=CARTESIAN_POINT('',(24.,9.,1.));
#13813=CARTESIAN_POINT('',(24.,9.,1.));
#13814=CARTESIAN_POINT('',(24.,9.,0.));
#13815=CARTESIAN_POINT('Origin',(24.,-18.,0.));
#13816=CARTESIAN_POINT('',(24.,-18.,0.));
#13817=CARTESIAN_POINT('',(24.,-18.,0.));
#13818=CARTESIAN_POINT('',(24.,-18.,1.));
#13819=CARTESIAN_POINT('',(24.,-18.,1.));
#13820=CARTESIAN_POINT('',(24.,-18.,0.));
#13821=CARTESIAN_POINT('Origin',(-8.,-18.,0.));
#13822=CARTESIAN_POINT('',(-8.,-18.,0.));
#13823=CARTESIAN_POINT('',(-8.,-18.,0.));
#13824=CARTESIAN_POINT('',(-8.,-18.,1.));
#13825=CARTESIAN_POINT('',(-8.,-18.,1.));
#13826=CARTESIAN_POINT('',(-8.,-18.,0.));
#13827=CARTESIAN_POINT('Origin',(-8.,9.,0.));
#13828=CARTESIAN_POINT('',(-8.,9.,0.));
#13829=CARTESIAN_POINT('',(-8.,9.,1.));
#13830=CARTESIAN_POINT('Origin',(8.,-4.5,1.));
#13831=CARTESIAN_POINT('Origin',(8.,-4.5,0.));
#17203=UNCERTAINTY_MEASURE_WITH_UNIT(LENGTH_MEASURE(0.001),#17323,
'DISTANCE_ACCURACY_VALUE',
'Maximum model space distance between geometric entities at asserted c
onnectivities');
#17261=UNCERTAINTY_MEASURE_WITH_UNIT(LENGTH_MEASURE(0.001),#17323,
'DISTANCE_ACCURACY_VALUE',
'Maximum model space distance between geometric entities at asserted c
onnectivities');
#17264=(
GEOMETRIC_REPRESENTATION_CONTEXT(3)
GLOBAL_UNCERTAINTY_ASSIGNED_CONTEXT((#17203))
GLOBAL_UNIT_ASSIGNED_CONTEXT((#17323,#17325,#17326))
REPRESENTATION_CONTEXT('','3D')
);
#17322=(
GEOMETRIC_REPRESENTATION_CONTEXT(3)
GLOBAL_UNCERTAINTY_ASSIGNED_CONTEXT((#17261))
GLOBAL_UNIT_ASSIGNED_CONTEXT((#17323,#17325,#17326))
REPRESENTATION_CONTEXT('','3D')
);
#17323=(
LENGTH_UNIT()
NAMED_UNIT(*)
SI_UNIT(.CENTI.,.METRE.)
);
#17325=(
NAMED_UNIT(*)
PLANE_ANGLE_UNIT()
SI_UNIT($,.RADIAN.)
);
#17326=(
NAMED_UNIT(*)
SI_UNIT($,.STERADIAN.)
SOLID_ANGLE_UNIT()
);
#17329=SHAPE_DEFINITION_REPRESENTATION(#17389,#17560);
#17389=PRODUCT_DEFINITION_SHAPE('',$,#17621);
#17560=SHAPE_REPRESENTATION('',(#9687),#17264);
#17618=PRODUCT_DEFINITION_CONTEXT('part definition',#17800,'design');
#17621=PRODUCT_DEFINITION('Base','Base',#17681,#17618);
#17681=PRODUCT_DEFINITION_FORMATION('',$,#17804);
#17800=APPLICATION_CONTEXT(
'Core Data for Automotive Mechanical Design Process');
#17801=PRODUCT_CONTEXT('part definition',#17800,'mechanical');
#17804=PRODUCT('Base','Base','Base',(#17801));
#17904=COLOUR_RGB('Dark Blue',0.08,0.2,0.34);
#17905=FILL_AREA_STYLE_COLOUR('',#17904);
#17906=FILL_AREA_STYLE('',(#17905));
#17907=SURFACE_STYLE_FILL_AREA(#17906);
#17908=SURFACE_SIDE_STYLE('',(#17907));
#17909=SURFACE_STYLE_USAGE(.BOTH.,#17908);
#17910=PRESENTATION_STYLE_ASSIGNMENT((#17909));
ENDSEC;
END-ISO-10303-21;
